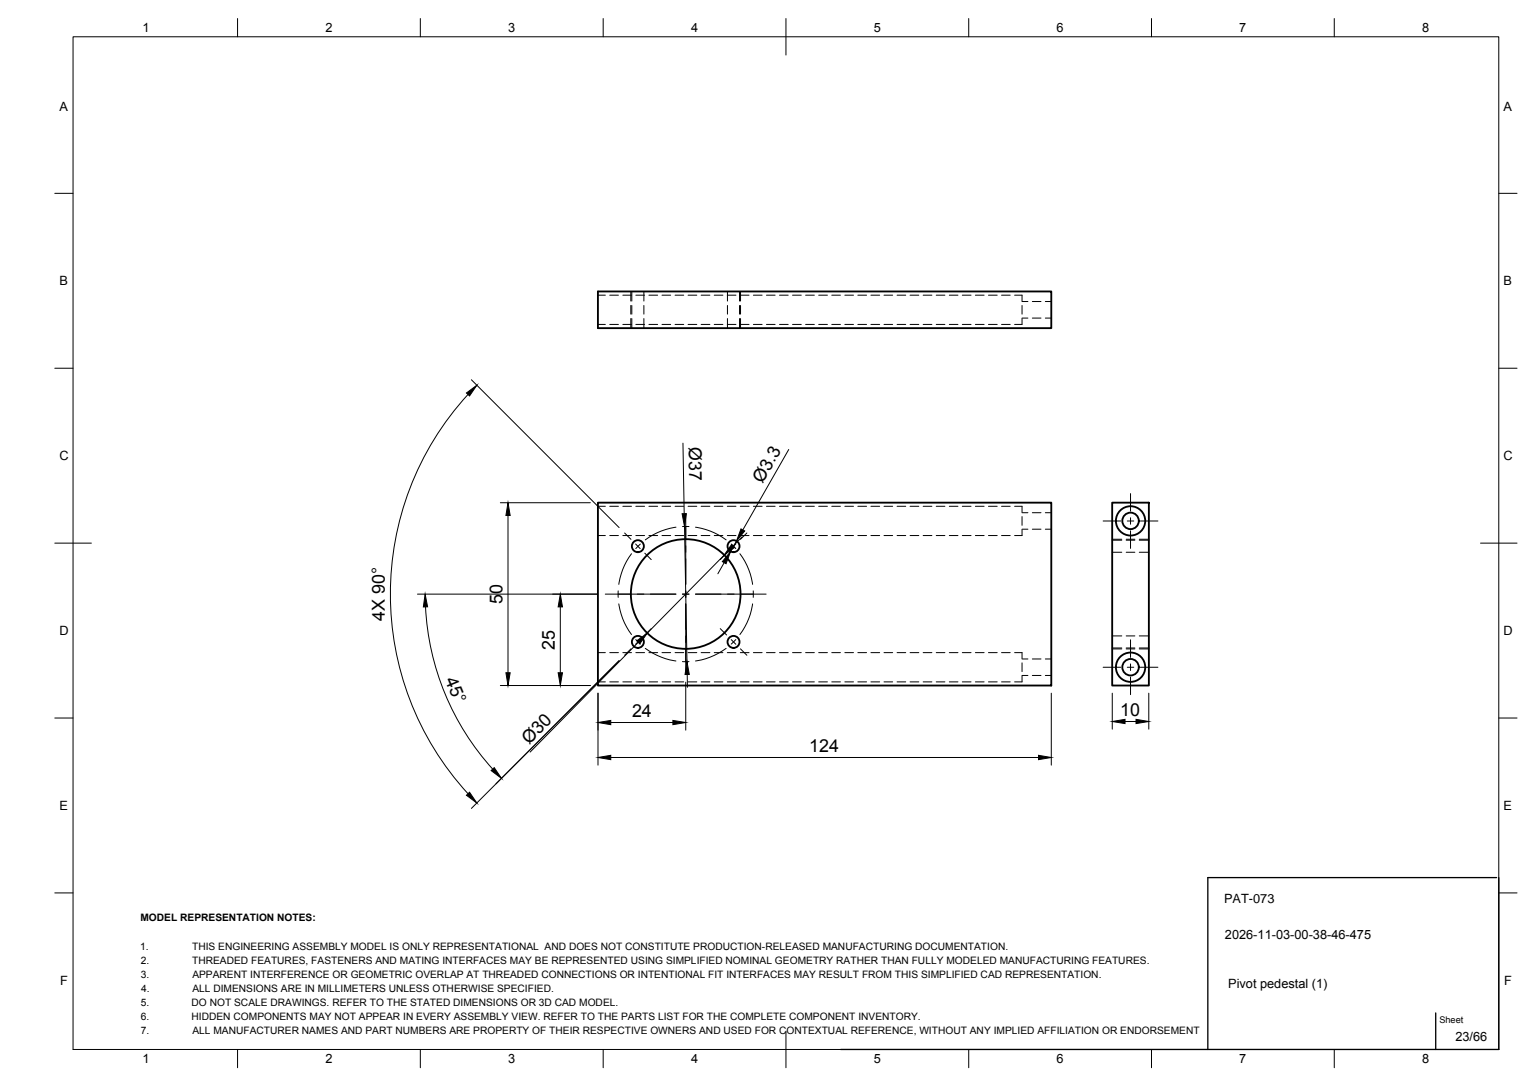
ISO-10303-21;
HEADER;
/* Generated by software containing ST-Developer
 * from STEP Tools, Inc. (www.steptools.com) 
 */

FILE_DESCRIPTION(
/* description */ ('Manual piston pump'),
/* implementation_level */ '2;1');

FILE_NAME(
/* name */ 'Pivot pedestal (1).step',
/* time_stamp */ '2026-11-02T16:54:23-08:00',
/* author */ (''),
/* organization */ (''),
/* preprocessor_version */ 'ST-DEVELOPER v20.2',
/* originating_system */ 'Autodesk Translation Framework v15.17.0.0',
/* authorisation */ '');

FILE_SCHEMA (('AUTOMOTIVE_DESIGN { 1 0 10303 214 3 1 1 }'));
ENDSEC;

DATA;
#10=MECHANICAL_DESIGN_GEOMETRIC_PRESENTATION_REPRESENTATION('',(#710),#19043);
#584=SHAPE_REPRESENTATION_RELATIONSHIP('SRR','None',#19330,#647);
#647=ADVANCED_BREP_SHAPE_REPRESENTATION('',(#780),#18997);
#710=STYLED_ITEM('',(#19661),#780);
#780=MANIFOLD_SOLID_BREP('Body1',#9496);
#930=FACE_BOUND('',#2197,.T.);
#931=FACE_BOUND('',#2201,.T.);
#932=FACE_BOUND('',#2205,.T.);
#933=FACE_BOUND('',#2206,.T.);
#934=FACE_BOUND('',#2209,.T.);
#935=FACE_BOUND('',#2210,.T.);
#936=FACE_BOUND('',#2213,.T.);
#937=FACE_BOUND('',#2214,.T.);
#938=FACE_BOUND('',#2215,.T.);
#939=FACE_BOUND('',#2216,.T.);
#940=FACE_BOUND('',#2217,.T.);
#941=FACE_BOUND('',#2219,.T.);
#942=FACE_BOUND('',#2220,.T.);
#943=FACE_BOUND('',#2221,.T.);
#944=FACE_BOUND('',#2222,.T.);
#945=FACE_BOUND('',#2223,.T.);
#1174=CYLINDRICAL_SURFACE('',#10669,0.164999999999999);
#1175=CYLINDRICAL_SURFACE('',#10672,0.164999999999999);
#1176=CYLINDRICAL_SURFACE('',#10675,0.164999999999999);
#1177=CYLINDRICAL_SURFACE('',#10678,0.164999999999999);
#1178=CYLINDRICAL_SURFACE('',#10681,0.4);
#1179=CYLINDRICAL_SURFACE('',#10686,0.225);
#1180=CYLINDRICAL_SURFACE('',#10688,0.4);
#1181=CYLINDRICAL_SURFACE('',#10693,0.225);
#1182=CYLINDRICAL_SURFACE('',#10695,1.5);
#1513=FACE_OUTER_BOUND('',#2191,.T.);
#1514=FACE_OUTER_BOUND('',#2192,.T.);
#1515=FACE_OUTER_BOUND('',#2193,.T.);
#1516=FACE_OUTER_BOUND('',#2194,.T.);
#1517=FACE_OUTER_BOUND('',#2195,.T.);
#1518=FACE_OUTER_BOUND('',#2196,.T.);
#1519=FACE_OUTER_BOUND('',#2198,.T.);
#1520=FACE_OUTER_BOUND('',#2199,.T.);
#1521=FACE_OUTER_BOUND('',#2200,.T.);
#1522=FACE_OUTER_BOUND('',#2202,.T.);
#1523=FACE_OUTER_BOUND('',#2203,.T.);
#1524=FACE_OUTER_BOUND('',#2204,.T.);
#1525=FACE_OUTER_BOUND('',#2207,.T.);
#1526=FACE_OUTER_BOUND('',#2208,.T.);
#1527=FACE_OUTER_BOUND('',#2211,.T.);
#1528=FACE_OUTER_BOUND('',#2212,.T.);
#1529=FACE_OUTER_BOUND('',#2218,.T.);
#2191=EDGE_LOOP('',(#7171,#7172,#7173,#7174));
#2192=EDGE_LOOP('',(#7175,#7176,#7177,#7178));
#2193=EDGE_LOOP('',(#7179,#7180,#7181,#7182));
#2194=EDGE_LOOP('',(#7183,#7184,#7185,#7186));
#2195=EDGE_LOOP('',(#7187,#7188,#7189,#7190));
#2196=EDGE_LOOP('',(#7191));
#2197=EDGE_LOOP('',(#7192));
#2198=EDGE_LOOP('',(#7193,#7194,#7195,#7196));
#2199=EDGE_LOOP('',(#7197,#7198,#7199,#7200));
#2200=EDGE_LOOP('',(#7201));
#2201=EDGE_LOOP('',(#7202));
#2202=EDGE_LOOP('',(#7203,#7204,#7205,#7206));
#2203=EDGE_LOOP('',(#7207,#7208,#7209,#7210));
#2204=EDGE_LOOP('',(#7211,#7212,#7213,#7214));
#2205=EDGE_LOOP('',(#7215));
#2206=EDGE_LOOP('',(#7216));
#2207=EDGE_LOOP('',(#7217,#7218,#7219,#7220));
#2208=EDGE_LOOP('',(#7221,#7222,#7223,#7224));
#2209=EDGE_LOOP('',(#7225));
#2210=EDGE_LOOP('',(#7226));
#2211=EDGE_LOOP('',(#7227,#7228,#7229,#7230));
#2212=EDGE_LOOP('',(#7231,#7232,#7233,#7234));
#2213=EDGE_LOOP('',(#7235));
#2214=EDGE_LOOP('',(#7236));
#2215=EDGE_LOOP('',(#7237));
#2216=EDGE_LOOP('',(#7238));
#2217=EDGE_LOOP('',(#7239));
#2218=EDGE_LOOP('',(#7240,#7241,#7242,#7243));
#2219=EDGE_LOOP('',(#7244));
#2220=EDGE_LOOP('',(#7245));
#2221=EDGE_LOOP('',(#7246));
#2222=EDGE_LOOP('',(#7247));
#2223=EDGE_LOOP('',(#7248));
#2843=CIRCLE('',#10670,0.164999999999999);
#2844=CIRCLE('',#10671,0.164999999999999);
#2845=CIRCLE('',#10673,0.164999999999999);
#2846=CIRCLE('',#10674,0.164999999999999);
#2847=CIRCLE('',#10676,0.164999999999999);
#2848=CIRCLE('',#10677,0.164999999999999);
#2849=CIRCLE('',#10679,0.164999999999999);
#2850=CIRCLE('',#10680,0.164999999999999);
#2851=CIRCLE('',#10682,0.4);
#2852=CIRCLE('',#10683,0.4);
#2853=CIRCLE('',#10685,0.225);
#2854=CIRCLE('',#10687,0.225);
#2855=CIRCLE('',#10689,0.4);
#2856=CIRCLE('',#10690,0.4);
#2857=CIRCLE('',#10692,0.225);
#2858=CIRCLE('',#10694,0.225);
#2859=CIRCLE('',#10696,1.5);
#2860=CIRCLE('',#10697,1.5);
#3401=LINE('',#15672,#4005);
#3402=LINE('',#15678,#4006);
#3403=LINE('',#15684,#4007);
#3404=LINE('',#15690,#4008);
#3405=LINE('',#15696,#4009);
#3406=LINE('',#15704,#4010);
#3407=LINE('',#15709,#4011);
#3408=LINE('',#15717,#4012);
#3409=LINE('',#15722,#4013);
#3410=LINE('',#15727,#4014);
#3411=LINE('',#15729,#4015);
#3412=LINE('',#15731,#4016);
#3413=LINE('',#15732,#4017);
#3414=LINE('',#15735,#4018);
#3415=LINE('',#15737,#4019);
#3416=LINE('',#15738,#4020);
#3417=LINE('',#15741,#4021);
#3418=LINE('',#15743,#4022);
#3419=LINE('',#15744,#4023);
#3420=LINE('',#15746,#4024);
#3421=LINE('',#15747,#4025);
#4005=VECTOR('',#12605,0.164999999999999);
#4006=VECTOR('',#12612,0.164999999999999);
#4007=VECTOR('',#12619,0.164999999999999);
#4008=VECTOR('',#12626,0.164999999999999);
#4009=VECTOR('',#12633,0.4);
#4010=VECTOR('',#12644,0.225);
#4011=VECTOR('',#12649,0.4);
#4012=VECTOR('',#12660,0.225);
#4013=VECTOR('',#12665,1.5);
#4014=VECTOR('',#12670,1.);
#4015=VECTOR('',#12671,1.);
#4016=VECTOR('',#12672,1.);
#4017=VECTOR('',#12673,1.);
#4018=VECTOR('',#12676,1.);
#4019=VECTOR('',#12677,1.);
#4020=VECTOR('',#12678,1.);
#4021=VECTOR('',#12681,1.);
#4022=VECTOR('',#12682,1.);
#4023=VECTOR('',#12683,1.);
#4024=VECTOR('',#12686,1.);
#4025=VECTOR('',#12687,1.);
#4650=VERTEX_POINT('',#15669);
#4651=VERTEX_POINT('',#15671);
#4652=VERTEX_POINT('',#15675);
#4653=VERTEX_POINT('',#15677);
#4654=VERTEX_POINT('',#15681);
#4655=VERTEX_POINT('',#15683);
#4656=VERTEX_POINT('',#15687);
#4657=VERTEX_POINT('',#15689);
#4658=VERTEX_POINT('',#15693);
#4659=VERTEX_POINT('',#15695);
#4660=VERTEX_POINT('',#15699);
#4661=VERTEX_POINT('',#15702);
#4662=VERTEX_POINT('',#15706);
#4663=VERTEX_POINT('',#15708);
#4664=VERTEX_POINT('',#15712);
#4665=VERTEX_POINT('',#15715);
#4666=VERTEX_POINT('',#15719);
#4667=VERTEX_POINT('',#15721);
#4668=VERTEX_POINT('',#15725);
#4669=VERTEX_POINT('',#15726);
#4670=VERTEX_POINT('',#15728);
#4671=VERTEX_POINT('',#15730);
#4672=VERTEX_POINT('',#15734);
#4673=VERTEX_POINT('',#15736);
#4674=VERTEX_POINT('',#15740);
#4675=VERTEX_POINT('',#15742);
#5572=EDGE_CURVE('',#4650,#4650,#2843,.T.);
#5573=EDGE_CURVE('',#4650,#4651,#3401,.T.);
#5574=EDGE_CURVE('',#4651,#4651,#2844,.T.);
#5575=EDGE_CURVE('',#4652,#4652,#2845,.T.);
#5576=EDGE_CURVE('',#4652,#4653,#3402,.T.);
#5577=EDGE_CURVE('',#4653,#4653,#2846,.T.);
#5578=EDGE_CURVE('',#4654,#4654,#2847,.T.);
#5579=EDGE_CURVE('',#4654,#4655,#3403,.T.);
#5580=EDGE_CURVE('',#4655,#4655,#2848,.T.);
#5581=EDGE_CURVE('',#4656,#4656,#2849,.T.);
#5582=EDGE_CURVE('',#4656,#4657,#3404,.T.);
#5583=EDGE_CURVE('',#4657,#4657,#2850,.T.);
#5584=EDGE_CURVE('',#4658,#4658,#2851,.T.);
#5585=EDGE_CURVE('',#4658,#4659,#3405,.T.);
#5586=EDGE_CURVE('',#4659,#4659,#2852,.T.);
#5587=EDGE_CURVE('',#4660,#4660,#2853,.T.);
#5588=EDGE_CURVE('',#4661,#4661,#2854,.T.);
#5589=EDGE_CURVE('',#4661,#4660,#3406,.T.);
#5590=EDGE_CURVE('',#4662,#4662,#2855,.T.);
#5591=EDGE_CURVE('',#4662,#4663,#3407,.T.);
#5592=EDGE_CURVE('',#4663,#4663,#2856,.T.);
#5593=EDGE_CURVE('',#4664,#4664,#2857,.T.);
#5594=EDGE_CURVE('',#4665,#4665,#2858,.T.);
#5595=EDGE_CURVE('',#4665,#4664,#3408,.T.);
#5596=EDGE_CURVE('',#4666,#4666,#2859,.T.);
#5597=EDGE_CURVE('',#4666,#4667,#3409,.T.);
#5598=EDGE_CURVE('',#4667,#4667,#2860,.T.);
#5599=EDGE_CURVE('',#4668,#4669,#3410,.T.);
#5600=EDGE_CURVE('',#4669,#4670,#3411,.T.);
#5601=EDGE_CURVE('',#4671,#4670,#3412,.T.);
#5602=EDGE_CURVE('',#4668,#4671,#3413,.T.);
#5603=EDGE_CURVE('',#4672,#4668,#3414,.T.);
#5604=EDGE_CURVE('',#4673,#4671,#3415,.T.);
#5605=EDGE_CURVE('',#4672,#4673,#3416,.T.);
#5606=EDGE_CURVE('',#4674,#4672,#3417,.T.);
#5607=EDGE_CURVE('',#4675,#4673,#3418,.T.);
#5608=EDGE_CURVE('',#4674,#4675,#3419,.T.);
#5609=EDGE_CURVE('',#4669,#4674,#3420,.T.);
#5610=EDGE_CURVE('',#4670,#4675,#3421,.T.);
#7171=ORIENTED_EDGE('',*,*,#5572,.F.);
#7172=ORIENTED_EDGE('',*,*,#5573,.T.);
#7173=ORIENTED_EDGE('',*,*,#5574,.F.);
#7174=ORIENTED_EDGE('',*,*,#5573,.F.);
#7175=ORIENTED_EDGE('',*,*,#5575,.F.);
#7176=ORIENTED_EDGE('',*,*,#5576,.T.);
#7177=ORIENTED_EDGE('',*,*,#5577,.F.);
#7178=ORIENTED_EDGE('',*,*,#5576,.F.);
#7179=ORIENTED_EDGE('',*,*,#5578,.F.);
#7180=ORIENTED_EDGE('',*,*,#5579,.T.);
#7181=ORIENTED_EDGE('',*,*,#5580,.F.);
#7182=ORIENTED_EDGE('',*,*,#5579,.F.);
#7183=ORIENTED_EDGE('',*,*,#5581,.F.);
#7184=ORIENTED_EDGE('',*,*,#5582,.T.);
#7185=ORIENTED_EDGE('',*,*,#5583,.F.);
#7186=ORIENTED_EDGE('',*,*,#5582,.F.);
#7187=ORIENTED_EDGE('',*,*,#5584,.F.);
#7188=ORIENTED_EDGE('',*,*,#5585,.T.);
#7189=ORIENTED_EDGE('',*,*,#5586,.F.);
#7190=ORIENTED_EDGE('',*,*,#5585,.F.);
#7191=ORIENTED_EDGE('',*,*,#5584,.T.);
#7192=ORIENTED_EDGE('',*,*,#5587,.F.);
#7193=ORIENTED_EDGE('',*,*,#5588,.F.);
#7194=ORIENTED_EDGE('',*,*,#5589,.T.);
#7195=ORIENTED_EDGE('',*,*,#5587,.T.);
#7196=ORIENTED_EDGE('',*,*,#5589,.F.);
#7197=ORIENTED_EDGE('',*,*,#5590,.F.);
#7198=ORIENTED_EDGE('',*,*,#5591,.T.);
#7199=ORIENTED_EDGE('',*,*,#5592,.F.);
#7200=ORIENTED_EDGE('',*,*,#5591,.F.);
#7201=ORIENTED_EDGE('',*,*,#5590,.T.);
#7202=ORIENTED_EDGE('',*,*,#5593,.F.);
#7203=ORIENTED_EDGE('',*,*,#5594,.F.);
#7204=ORIENTED_EDGE('',*,*,#5595,.T.);
#7205=ORIENTED_EDGE('',*,*,#5593,.T.);
#7206=ORIENTED_EDGE('',*,*,#5595,.F.);
#7207=ORIENTED_EDGE('',*,*,#5596,.F.);
#7208=ORIENTED_EDGE('',*,*,#5597,.T.);
#7209=ORIENTED_EDGE('',*,*,#5598,.F.);
#7210=ORIENTED_EDGE('',*,*,#5597,.F.);
#7211=ORIENTED_EDGE('',*,*,#5599,.T.);
#7212=ORIENTED_EDGE('',*,*,#5600,.T.);
#7213=ORIENTED_EDGE('',*,*,#5601,.F.);
#7214=ORIENTED_EDGE('',*,*,#5602,.F.);
#7215=ORIENTED_EDGE('',*,*,#5586,.T.);
#7216=ORIENTED_EDGE('',*,*,#5592,.T.);
#7217=ORIENTED_EDGE('',*,*,#5603,.T.);
#7218=ORIENTED_EDGE('',*,*,#5602,.T.);
#7219=ORIENTED_EDGE('',*,*,#5604,.F.);
#7220=ORIENTED_EDGE('',*,*,#5605,.F.);
#7221=ORIENTED_EDGE('',*,*,#5606,.T.);
#7222=ORIENTED_EDGE('',*,*,#5605,.T.);
#7223=ORIENTED_EDGE('',*,*,#5607,.F.);
#7224=ORIENTED_EDGE('',*,*,#5608,.F.);
#7225=ORIENTED_EDGE('',*,*,#5588,.T.);
#7226=ORIENTED_EDGE('',*,*,#5594,.T.);
#7227=ORIENTED_EDGE('',*,*,#5609,.T.);
#7228=ORIENTED_EDGE('',*,*,#5608,.T.);
#7229=ORIENTED_EDGE('',*,*,#5610,.F.);
#7230=ORIENTED_EDGE('',*,*,#5600,.F.);
#7231=ORIENTED_EDGE('',*,*,#5610,.T.);
#7232=ORIENTED_EDGE('',*,*,#5607,.T.);
#7233=ORIENTED_EDGE('',*,*,#5604,.T.);
#7234=ORIENTED_EDGE('',*,*,#5601,.T.);
#7235=ORIENTED_EDGE('',*,*,#5598,.T.);
#7236=ORIENTED_EDGE('',*,*,#5583,.T.);
#7237=ORIENTED_EDGE('',*,*,#5580,.T.);
#7238=ORIENTED_EDGE('',*,*,#5577,.T.);
#7239=ORIENTED_EDGE('',*,*,#5574,.T.);
#7240=ORIENTED_EDGE('',*,*,#5609,.F.);
#7241=ORIENTED_EDGE('',*,*,#5599,.F.);
#7242=ORIENTED_EDGE('',*,*,#5603,.F.);
#7243=ORIENTED_EDGE('',*,*,#5606,.F.);
#7244=ORIENTED_EDGE('',*,*,#5596,.T.);
#7245=ORIENTED_EDGE('',*,*,#5581,.T.);
#7246=ORIENTED_EDGE('',*,*,#5578,.T.);
#7247=ORIENTED_EDGE('',*,*,#5575,.T.);
#7248=ORIENTED_EDGE('',*,*,#5572,.T.);
#8700=PLANE('',#10684);
#8701=PLANE('',#10691);
#8702=PLANE('',#10698);
#8703=PLANE('',#10699);
#8704=PLANE('',#10700);
#8705=PLANE('',#10701);
#8706=PLANE('',#10702);
#8707=PLANE('',#10703);
#9118=ADVANCED_FACE('',(#1513),#1174,.F.);
#9119=ADVANCED_FACE('',(#1514),#1175,.F.);
#9120=ADVANCED_FACE('',(#1515),#1176,.F.);
#9121=ADVANCED_FACE('',(#1516),#1177,.F.);
#9122=ADVANCED_FACE('',(#1517),#1178,.F.);
#9123=ADVANCED_FACE('',(#1518,#930),#8700,.T.);
#9124=ADVANCED_FACE('',(#1519),#1179,.F.);
#9125=ADVANCED_FACE('',(#1520),#1180,.F.);
#9126=ADVANCED_FACE('',(#1521,#931),#8701,.T.);
#9127=ADVANCED_FACE('',(#1522),#1181,.F.);
#9128=ADVANCED_FACE('',(#1523),#1182,.F.);
#9129=ADVANCED_FACE('',(#1524,#932,#933),#8702,.T.);
#9130=ADVANCED_FACE('',(#1525),#8703,.T.);
#9131=ADVANCED_FACE('',(#1526,#934,#935),#8704,.T.);
#9132=ADVANCED_FACE('',(#1527),#8705,.T.);
#9133=ADVANCED_FACE('',(#1528,#936,#937,#938,#939,#940),#8706,.T.);
#9134=ADVANCED_FACE('',(#1529,#941,#942,#943,#944,#945),#8707,.F.);
#9496=CLOSED_SHELL('',(#9118,#9119,#9120,#9121,#9122,#9123,#9124,#9125,
#9126,#9127,#9128,#9129,#9130,#9131,#9132,#9133,#9134));
#10668=AXIS2_PLACEMENT_3D('',#15667,#12599,#12600);
#10669=AXIS2_PLACEMENT_3D('',#15668,#12601,#12602);
#10670=AXIS2_PLACEMENT_3D('',#15670,#12603,#12604);
#10671=AXIS2_PLACEMENT_3D('',#15673,#12606,#12607);
#10672=AXIS2_PLACEMENT_3D('',#15674,#12608,#12609);
#10673=AXIS2_PLACEMENT_3D('',#15676,#12610,#12611);
#10674=AXIS2_PLACEMENT_3D('',#15679,#12613,#12614);
#10675=AXIS2_PLACEMENT_3D('',#15680,#12615,#12616);
#10676=AXIS2_PLACEMENT_3D('',#15682,#12617,#12618);
#10677=AXIS2_PLACEMENT_3D('',#15685,#12620,#12621);
#10678=AXIS2_PLACEMENT_3D('',#15686,#12622,#12623);
#10679=AXIS2_PLACEMENT_3D('',#15688,#12624,#12625);
#10680=AXIS2_PLACEMENT_3D('',#15691,#12627,#12628);
#10681=AXIS2_PLACEMENT_3D('',#15692,#12629,#12630);
#10682=AXIS2_PLACEMENT_3D('',#15694,#12631,#12632);
#10683=AXIS2_PLACEMENT_3D('',#15697,#12634,#12635);
#10684=AXIS2_PLACEMENT_3D('',#15698,#12636,#12637);
#10685=AXIS2_PLACEMENT_3D('',#15700,#12638,#12639);
#10686=AXIS2_PLACEMENT_3D('',#15701,#12640,#12641);
#10687=AXIS2_PLACEMENT_3D('',#15703,#12642,#12643);
#10688=AXIS2_PLACEMENT_3D('',#15705,#12645,#12646);
#10689=AXIS2_PLACEMENT_3D('',#15707,#12647,#12648);
#10690=AXIS2_PLACEMENT_3D('',#15710,#12650,#12651);
#10691=AXIS2_PLACEMENT_3D('',#15711,#12652,#12653);
#10692=AXIS2_PLACEMENT_3D('',#15713,#12654,#12655);
#10693=AXIS2_PLACEMENT_3D('',#15714,#12656,#12657);
#10694=AXIS2_PLACEMENT_3D('',#15716,#12658,#12659);
#10695=AXIS2_PLACEMENT_3D('',#15718,#12661,#12662);
#10696=AXIS2_PLACEMENT_3D('',#15720,#12663,#12664);
#10697=AXIS2_PLACEMENT_3D('',#15723,#12666,#12667);
#10698=AXIS2_PLACEMENT_3D('',#15724,#12668,#12669);
#10699=AXIS2_PLACEMENT_3D('',#15733,#12674,#12675);
#10700=AXIS2_PLACEMENT_3D('',#15739,#12679,#12680);
#10701=AXIS2_PLACEMENT_3D('',#15745,#12684,#12685);
#10702=AXIS2_PLACEMENT_3D('',#15748,#12688,#12689);
#10703=AXIS2_PLACEMENT_3D('',#15749,#12690,#12691);
#12599=DIRECTION('axis',(0.,0.,1.));
#12600=DIRECTION('refdir',(1.,0.,0.));
#12601=DIRECTION('center_axis',(1.,0.,0.));
#12602=DIRECTION('ref_axis',(0.,0.,-1.));
#12603=DIRECTION('center_axis',(1.,0.,0.));
#12604=DIRECTION('ref_axis',(0.,0.,-1.));
#12605=DIRECTION('',(1.,0.,0.));
#12606=DIRECTION('center_axis',(-1.,0.,0.));
#12607=DIRECTION('ref_axis',(0.,0.,-1.));
#12608=DIRECTION('center_axis',(1.,0.,0.));
#12609=DIRECTION('ref_axis',(0.,0.,-1.));
#12610=DIRECTION('center_axis',(1.,0.,0.));
#12611=DIRECTION('ref_axis',(0.,0.,-1.));
#12612=DIRECTION('',(1.,0.,0.));
#12613=DIRECTION('center_axis',(-1.,0.,0.));
#12614=DIRECTION('ref_axis',(0.,0.,-1.));
#12615=DIRECTION('center_axis',(1.,0.,0.));
#12616=DIRECTION('ref_axis',(0.,0.,-1.));
#12617=DIRECTION('center_axis',(1.,0.,0.));
#12618=DIRECTION('ref_axis',(0.,0.,-1.));
#12619=DIRECTION('',(1.,0.,0.));
#12620=DIRECTION('center_axis',(-1.,0.,0.));
#12621=DIRECTION('ref_axis',(0.,0.,-1.));
#12622=DIRECTION('center_axis',(1.,0.,0.));
#12623=DIRECTION('ref_axis',(0.,0.,-1.));
#12624=DIRECTION('center_axis',(1.,0.,0.));
#12625=DIRECTION('ref_axis',(0.,0.,-1.));
#12626=DIRECTION('',(1.,0.,0.));
#12627=DIRECTION('center_axis',(-1.,0.,0.));
#12628=DIRECTION('ref_axis',(0.,0.,-1.));
#12629=DIRECTION('center_axis',(0.,0.,1.));
#12630=DIRECTION('ref_axis',(1.,0.,0.));
#12631=DIRECTION('center_axis',(0.,0.,1.));
#12632=DIRECTION('ref_axis',(1.,0.,0.));
#12633=DIRECTION('',(0.,0.,1.));
#12634=DIRECTION('center_axis',(0.,0.,-1.));
#12635=DIRECTION('ref_axis',(1.,0.,0.));
#12636=DIRECTION('center_axis',(0.,0.,1.));
#12637=DIRECTION('ref_axis',(1.,0.,0.));
#12638=DIRECTION('center_axis',(0.,0.,1.));
#12639=DIRECTION('ref_axis',(1.,0.,0.));
#12640=DIRECTION('center_axis',(0.,0.,1.));
#12641=DIRECTION('ref_axis',(1.,0.,0.));
#12642=DIRECTION('center_axis',(0.,0.,1.));
#12643=DIRECTION('ref_axis',(1.,0.,0.));
#12644=DIRECTION('',(0.,0.,1.));
#12645=DIRECTION('center_axis',(0.,0.,1.));
#12646=DIRECTION('ref_axis',(1.,0.,0.));
#12647=DIRECTION('center_axis',(0.,0.,1.));
#12648=DIRECTION('ref_axis',(1.,0.,0.));
#12649=DIRECTION('',(0.,0.,1.));
#12650=DIRECTION('center_axis',(0.,0.,-1.));
#12651=DIRECTION('ref_axis',(1.,0.,0.));
#12652=DIRECTION('center_axis',(0.,0.,1.));
#12653=DIRECTION('ref_axis',(1.,0.,0.));
#12654=DIRECTION('center_axis',(0.,0.,1.));
#12655=DIRECTION('ref_axis',(1.,0.,0.));
#12656=DIRECTION('center_axis',(0.,0.,1.));
#12657=DIRECTION('ref_axis',(1.,0.,0.));
#12658=DIRECTION('center_axis',(0.,0.,1.));
#12659=DIRECTION('ref_axis',(1.,0.,0.));
#12660=DIRECTION('',(0.,0.,1.));
#12661=DIRECTION('center_axis',(1.,0.,0.));
#12662=DIRECTION('ref_axis',(0.,0.,-1.));
#12663=DIRECTION('center_axis',(1.,0.,0.));
#12664=DIRECTION('ref_axis',(0.,0.,-1.));
#12665=DIRECTION('',(1.,0.,0.));
#12666=DIRECTION('center_axis',(-1.,0.,0.));
#12667=DIRECTION('ref_axis',(0.,0.,-1.));
#12668=DIRECTION('center_axis',(0.,0.,1.));
#12669=DIRECTION('ref_axis',(0.,-1.,0.));
#12670=DIRECTION('',(0.,-1.,0.));
#12671=DIRECTION('',(1.,0.,0.));
#12672=DIRECTION('',(0.,-1.,0.));
#12673=DIRECTION('',(1.,0.,0.));
#12674=DIRECTION('center_axis',(0.,1.,0.));
#12675=DIRECTION('ref_axis',(0.,0.,1.));
#12676=DIRECTION('',(0.,0.,1.));
#12677=DIRECTION('',(0.,0.,1.));
#12678=DIRECTION('',(1.,0.,0.));
#12679=DIRECTION('center_axis',(0.,0.,-1.));
#12680=DIRECTION('ref_axis',(0.,1.,0.));
#12681=DIRECTION('',(0.,1.,0.));
#12682=DIRECTION('',(0.,1.,0.));
#12683=DIRECTION('',(1.,0.,0.));
#12684=DIRECTION('center_axis',(0.,-1.,0.));
#12685=DIRECTION('ref_axis',(0.,0.,-1.));
#12686=DIRECTION('',(0.,0.,-1.));
#12687=DIRECTION('',(0.,0.,-1.));
#12688=DIRECTION('center_axis',(1.,0.,0.));
#12689=DIRECTION('ref_axis',(0.,0.,-1.));
#12690=DIRECTION('center_axis',(1.,0.,0.));
#12691=DIRECTION('ref_axis',(0.,0.,-1.));
#15667=CARTESIAN_POINT('',(0.,0.,0.));
#15668=CARTESIAN_POINT('Origin',(2.9,-5.30814754519511,8.69185245480489));
#15669=CARTESIAN_POINT('',(3.,-5.30814754519511,8.85685245480489));
#15670=CARTESIAN_POINT('Origin',(3.,-5.30814754519511,8.69185245480489));
#15671=CARTESIAN_POINT('',(4.,-5.30814754519511,8.85685245480489));
#15672=CARTESIAN_POINT('',(2.9,-5.30814754519511,8.85685245480489));
#15673=CARTESIAN_POINT('Origin',(4.,-5.30814754519511,8.69185245480489));
#15674=CARTESIAN_POINT('Origin',(2.9,-5.30814754519511,11.3081475451951));
#15675=CARTESIAN_POINT('',(3.,-5.30814754519511,11.4731475451951));
#15676=CARTESIAN_POINT('Origin',(3.,-5.30814754519511,11.3081475451951));
#15677=CARTESIAN_POINT('',(4.,-5.30814754519511,11.4731475451951));
#15678=CARTESIAN_POINT('',(2.9,-5.30814754519511,11.4731475451951));
#15679=CARTESIAN_POINT('Origin',(4.,-5.30814754519511,11.3081475451951));
#15680=CARTESIAN_POINT('Origin',(2.9,-2.69185245480489,11.3081475451951));
#15681=CARTESIAN_POINT('',(3.,-2.69185245480489,11.4731475451951));
#15682=CARTESIAN_POINT('Origin',(3.,-2.69185245480489,11.3081475451951));
#15683=CARTESIAN_POINT('',(4.,-2.69185245480489,11.4731475451951));
#15684=CARTESIAN_POINT('',(2.9,-2.69185245480489,11.4731475451951));
#15685=CARTESIAN_POINT('Origin',(4.,-2.69185245480489,11.3081475451951));
#15686=CARTESIAN_POINT('Origin',(2.9,-2.69185245480489,8.69185245480489));
#15687=CARTESIAN_POINT('',(3.,-2.69185245480489,8.85685245480489));
#15688=CARTESIAN_POINT('Origin',(3.,-2.69185245480489,8.69185245480489));
#15689=CARTESIAN_POINT('',(4.,-2.69185245480489,8.85685245480489));
#15690=CARTESIAN_POINT('',(2.9,-2.69185245480489,8.85685245480489));
#15691=CARTESIAN_POINT('Origin',(4.,-2.69185245480489,8.69185245480489));
#15692=CARTESIAN_POINT('Origin',(3.5,-2.,0.8));
#15693=CARTESIAN_POINT('',(3.1,-2.,0.8));
#15694=CARTESIAN_POINT('Origin',(3.5,-2.,0.8));
#15695=CARTESIAN_POINT('',(3.1,-2.,12.4));
#15696=CARTESIAN_POINT('',(3.1,-2.,0.8));
#15697=CARTESIAN_POINT('Origin',(3.5,-2.,12.4));
#15698=CARTESIAN_POINT('Origin',(3.5,-2.,0.8));
#15699=CARTESIAN_POINT('',(3.275,-2.,0.8));
#15700=CARTESIAN_POINT('Origin',(3.5,-2.,0.8));
#15701=CARTESIAN_POINT('Origin',(3.5,-2.,-0.1));
#15702=CARTESIAN_POINT('',(3.275,-2.,0.));
#15703=CARTESIAN_POINT('Origin',(3.5,-2.,0.));
#15704=CARTESIAN_POINT('',(3.275,-2.,-0.1));
#15705=CARTESIAN_POINT('Origin',(3.5,-6.,0.8));
#15706=CARTESIAN_POINT('',(3.1,-6.,0.8));
#15707=CARTESIAN_POINT('Origin',(3.5,-6.,0.8));
#15708=CARTESIAN_POINT('',(3.1,-6.,12.4));
#15709=CARTESIAN_POINT('',(3.1,-6.,0.8));
#15710=CARTESIAN_POINT('Origin',(3.5,-6.,12.4));
#15711=CARTESIAN_POINT('Origin',(3.5,-6.,0.8));
#15712=CARTESIAN_POINT('',(3.275,-6.,0.8));
#15713=CARTESIAN_POINT('Origin',(3.5,-6.,0.8));
#15714=CARTESIAN_POINT('Origin',(3.5,-6.,-0.1));
#15715=CARTESIAN_POINT('',(3.275,-6.,0.));
#15716=CARTESIAN_POINT('Origin',(3.5,-6.,0.));
#15717=CARTESIAN_POINT('',(3.275,-6.,-0.1));
#15718=CARTESIAN_POINT('Origin',(2.9,-4.,10.));
#15719=CARTESIAN_POINT('',(3.,-4.,11.5));
#15720=CARTESIAN_POINT('Origin',(3.,-4.,10.));
#15721=CARTESIAN_POINT('',(4.,-4.,11.5));
#15722=CARTESIAN_POINT('',(2.9,-4.,11.5));
#15723=CARTESIAN_POINT('Origin',(4.,-4.,10.));
#15724=CARTESIAN_POINT('Origin',(3.,-1.5,12.4));
#15725=CARTESIAN_POINT('',(3.,-1.5,12.4));
#15726=CARTESIAN_POINT('',(3.,-6.5,12.4));
#15727=CARTESIAN_POINT('',(3.,-1.5,12.4));
#15728=CARTESIAN_POINT('',(4.,-6.5,12.4));
#15729=CARTESIAN_POINT('',(3.,-6.5,12.4));
#15730=CARTESIAN_POINT('',(4.,-1.5,12.4));
#15731=CARTESIAN_POINT('',(4.,-1.5,12.4));
#15732=CARTESIAN_POINT('',(3.,-1.5,12.4));
#15733=CARTESIAN_POINT('Origin',(3.,-1.5,0.));
#15734=CARTESIAN_POINT('',(3.,-1.5,0.));
#15735=CARTESIAN_POINT('',(3.,-1.5,0.));
#15736=CARTESIAN_POINT('',(4.,-1.5,0.));
#15737=CARTESIAN_POINT('',(4.,-1.5,0.));
#15738=CARTESIAN_POINT('',(3.,-1.5,0.));
#15739=CARTESIAN_POINT('Origin',(3.,-6.5,0.));
#15740=CARTESIAN_POINT('',(3.,-6.5,0.));
#15741=CARTESIAN_POINT('',(3.,-6.5,0.));
#15742=CARTESIAN_POINT('',(4.,-6.5,0.));
#15743=CARTESIAN_POINT('',(4.,-6.5,0.));
#15744=CARTESIAN_POINT('',(3.,-6.5,0.));
#15745=CARTESIAN_POINT('Origin',(3.,-6.5,12.4));
#15746=CARTESIAN_POINT('',(3.,-6.5,12.4));
#15747=CARTESIAN_POINT('',(4.,-6.5,12.4));
#15748=CARTESIAN_POINT('Origin',(4.,-4.,6.2));
#15749=CARTESIAN_POINT('Origin',(3.,-4.,6.2));
#18926=UNCERTAINTY_MEASURE_WITH_UNIT(LENGTH_MEASURE(0.001),#19044,
'DISTANCE_ACCURACY_VALUE',
'Maximum model space distance between geometric entities at asserted c
onnectivities');
#18972=UNCERTAINTY_MEASURE_WITH_UNIT(LENGTH_MEASURE(0.001),#19044,
'DISTANCE_ACCURACY_VALUE',
'Maximum model space distance between geometric entities at asserted c
onnectivities');
#18997=(
GEOMETRIC_REPRESENTATION_CONTEXT(3)
GLOBAL_UNCERTAINTY_ASSIGNED_CONTEXT((#18926))
GLOBAL_UNIT_ASSIGNED_CONTEXT((#19044,#19046,#19047))
REPRESENTATION_CONTEXT('','3D')
);
#19043=(
GEOMETRIC_REPRESENTATION_CONTEXT(3)
GLOBAL_UNCERTAINTY_ASSIGNED_CONTEXT((#18972))
GLOBAL_UNIT_ASSIGNED_CONTEXT((#19044,#19046,#19047))
REPRESENTATION_CONTEXT('','3D')
);
#19044=(
LENGTH_UNIT()
NAMED_UNIT(*)
SI_UNIT(.CENTI.,.METRE.)
);
#19046=(
NAMED_UNIT(*)
PLANE_ANGLE_UNIT()
SI_UNIT($,.RADIAN.)
);
#19047=(
NAMED_UNIT(*)
SI_UNIT($,.STERADIAN.)
SOLID_ANGLE_UNIT()
);
#19072=SHAPE_DEFINITION_REPRESENTATION(#19142,#19330);
#19142=PRODUCT_DEFINITION_SHAPE('',$,#19401);
#19330=SHAPE_REPRESENTATION('',(#10668),#18997);
#19376=PRODUCT_DEFINITION_CONTEXT('part definition',#19588,'design');
#19401=PRODUCT_DEFINITION('2026-11-03-00-38-46-475',
'Pivot pedestal (1)',#19471,#19376);
#19471=PRODUCT_DEFINITION_FORMATION('',$,#19614);
#19588=APPLICATION_CONTEXT(
'Core Data for Automotive Mechanical Design Process');
#19589=PRODUCT_CONTEXT('part definition',#19588,'mechanical');
#19614=PRODUCT('2026-11-03-00-38-46-475','Pivot pedestal (1)',
'Pivot pedestal',(#19589));
#19661=PRESENTATION_STYLE_ASSIGNMENT((#19667));
#19667=SURFACE_STYLE_USAGE(.BOTH.,#19673);
#19673=SURFACE_SIDE_STYLE('',(#19679));
#19679=SURFACE_STYLE_FILL_AREA(#19685);
#19685=FILL_AREA_STYLE('CAD Library Painted - Engineering blue',(#19691));
#19691=FILL_AREA_STYLE_COLOUR('CAD Library Painted - Engineering blue',
#19697);
#19697=COLOUR_RGB('CAD Library Painted - Engineering blue',0.12156862745098,
0.356862745098039,0.6);
ENDSEC;
END-ISO-10303-21;
